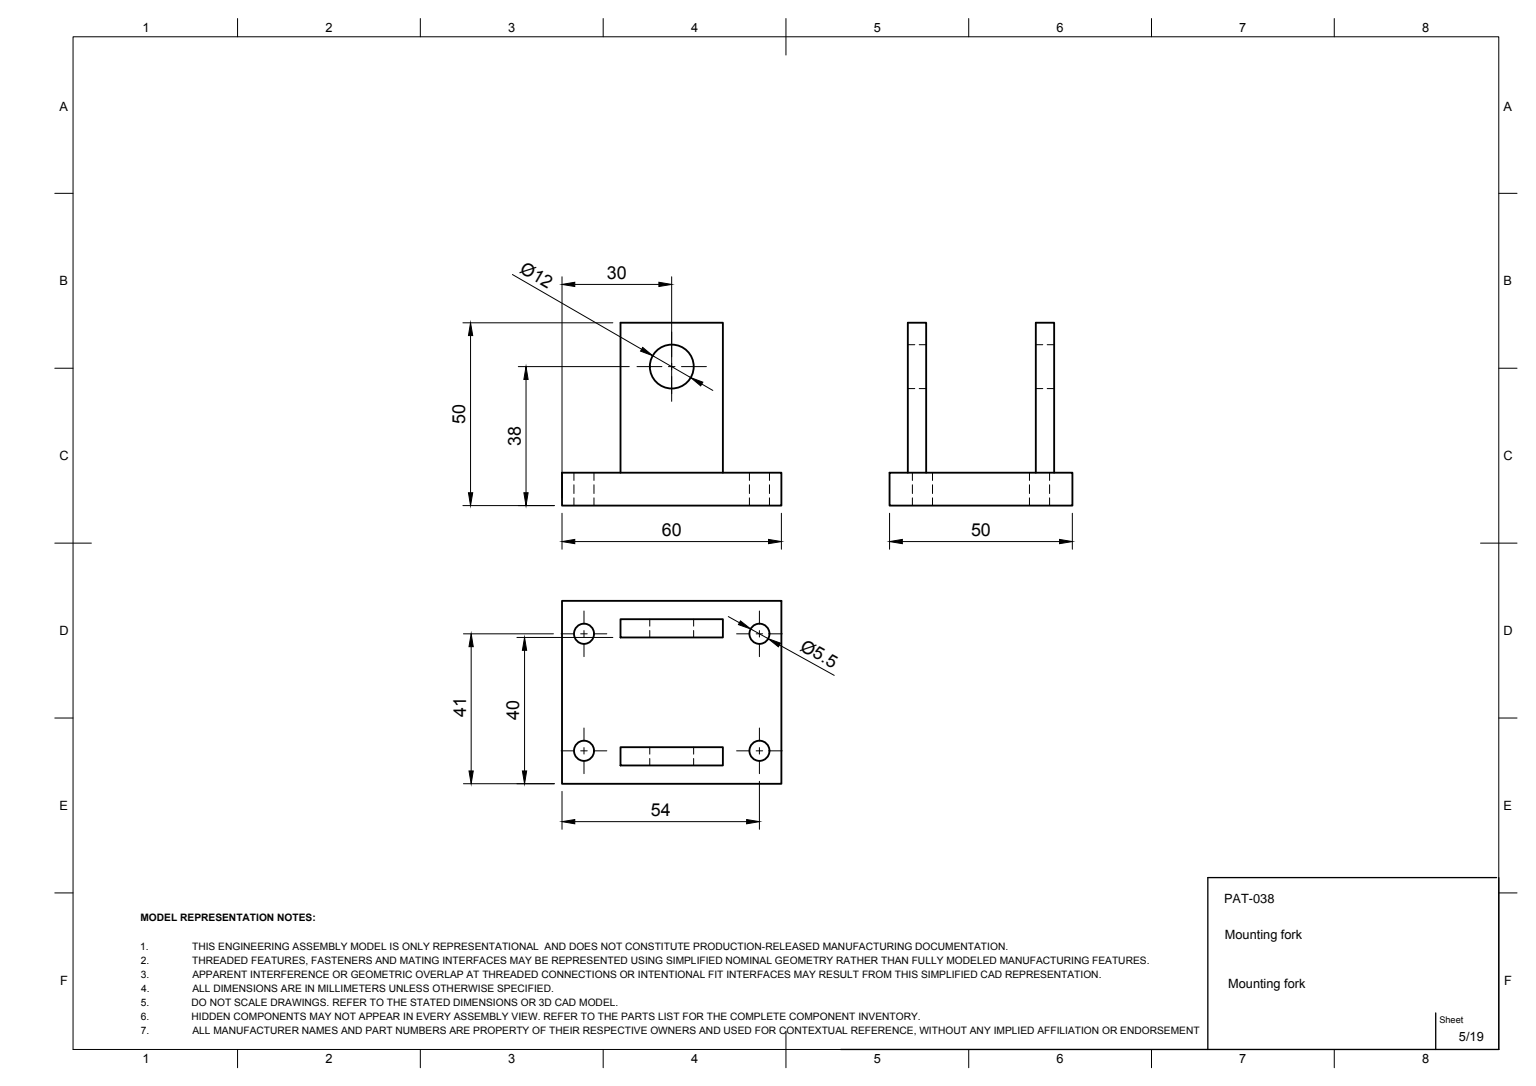
ISO-10303-21;
HEADER;
/* Generated by software containing ST-Developer
 * from STEP Tools, Inc. (www.steptools.com) 
 */

FILE_DESCRIPTION(
/* description */ ('Fork-mounted skate wheel'),
/* implementation_level */ '2;1');

FILE_NAME(
/* name */ 'Mounting fork.step',
/* time_stamp */ '2026-10-29T16:11:26-07:00',
/* author */ (''),
/* organization */ (''),
/* preprocessor_version */ 'ST-DEVELOPER v20.2',
/* originating_system */ 'Autodesk Translation Framework v15.17.0.0',
/* authorisation */ '');

FILE_SCHEMA (('AUTOMOTIVE_DESIGN { 1 0 10303 214 3 1 1 }'));
ENDSEC;

DATA;
#10=MECHANICAL_DESIGN_GEOMETRIC_PRESENTATION_REPRESENTATION('',(#146),#3688);
#122=SHAPE_REPRESENTATION_RELATIONSHIP('SRR','None',#3745,#134);
#134=ADVANCED_BREP_SHAPE_REPRESENTATION('',(#165),#3674);
#146=STYLED_ITEM('',(#3882),#165);
#165=MANIFOLD_SOLID_BREP('Body1',#1807);
#183=FACE_BOUND('',#396,.T.);
#184=FACE_BOUND('',#401,.T.);
#185=FACE_BOUND('',#403,.T.);
#186=FACE_BOUND('',#408,.T.);
#187=FACE_BOUND('',#414,.T.);
#188=FACE_BOUND('',#415,.T.);
#189=FACE_BOUND('',#416,.T.);
#190=FACE_BOUND('',#417,.T.);
#191=FACE_BOUND('',#418,.T.);
#192=FACE_BOUND('',#419,.T.);
#193=FACE_BOUND('',#421,.T.);
#194=FACE_BOUND('',#422,.T.);
#195=FACE_BOUND('',#423,.T.);
#196=FACE_BOUND('',#424,.T.);
#219=PLANE('',#1981);
#220=PLANE('',#1982);
#221=PLANE('',#1983);
#222=PLANE('',#1984);
#223=PLANE('',#1985);
#224=PLANE('',#1986);
#225=PLANE('',#1987);
#226=PLANE('',#1988);
#227=PLANE('',#1989);
#228=PLANE('',#1990);
#229=PLANE('',#1991);
#230=PLANE('',#1992);
#231=PLANE('',#1993);
#232=PLANE('',#1994);
#233=PLANE('',#1995);
#234=PLANE('',#1996);
#276=FACE_OUTER_BOUND('',#389,.T.);
#277=FACE_OUTER_BOUND('',#390,.T.);
#278=FACE_OUTER_BOUND('',#391,.T.);
#279=FACE_OUTER_BOUND('',#392,.T.);
#280=FACE_OUTER_BOUND('',#393,.T.);
#281=FACE_OUTER_BOUND('',#394,.T.);
#282=FACE_OUTER_BOUND('',#395,.T.);
#283=FACE_OUTER_BOUND('',#397,.T.);
#284=FACE_OUTER_BOUND('',#398,.T.);
#285=FACE_OUTER_BOUND('',#399,.T.);
#286=FACE_OUTER_BOUND('',#400,.T.);
#287=FACE_OUTER_BOUND('',#402,.T.);
#288=FACE_OUTER_BOUND('',#404,.T.);
#289=FACE_OUTER_BOUND('',#405,.T.);
#290=FACE_OUTER_BOUND('',#406,.T.);
#291=FACE_OUTER_BOUND('',#407,.T.);
#292=FACE_OUTER_BOUND('',#409,.T.);
#293=FACE_OUTER_BOUND('',#410,.T.);
#294=FACE_OUTER_BOUND('',#411,.T.);
#295=FACE_OUTER_BOUND('',#412,.T.);
#296=FACE_OUTER_BOUND('',#413,.T.);
#297=FACE_OUTER_BOUND('',#420,.T.);
#389=EDGE_LOOP('',(#1217,#1218,#1219,#1220));
#390=EDGE_LOOP('',(#1221,#1222,#1223,#1224));
#391=EDGE_LOOP('',(#1225,#1226,#1227,#1228));
#392=EDGE_LOOP('',(#1229,#1230,#1231,#1232));
#393=EDGE_LOOP('',(#1233,#1234,#1235,#1236));
#394=EDGE_LOOP('',(#1237,#1238,#1239,#1240));
#395=EDGE_LOOP('',(#1241,#1242,#1243,#1244));
#396=EDGE_LOOP('',(#1245));
#397=EDGE_LOOP('',(#1246,#1247,#1248,#1249));
#398=EDGE_LOOP('',(#1250,#1251,#1252,#1253));
#399=EDGE_LOOP('',(#1254,#1255,#1256,#1257));
#400=EDGE_LOOP('',(#1258,#1259,#1260,#1261));
#401=EDGE_LOOP('',(#1262));
#402=EDGE_LOOP('',(#1263,#1264,#1265,#1266));
#403=EDGE_LOOP('',(#1267));
#404=EDGE_LOOP('',(#1268,#1269,#1270,#1271));
#405=EDGE_LOOP('',(#1272,#1273,#1274,#1275));
#406=EDGE_LOOP('',(#1276,#1277,#1278,#1279));
#407=EDGE_LOOP('',(#1280,#1281,#1282,#1283));
#408=EDGE_LOOP('',(#1284));
#409=EDGE_LOOP('',(#1285,#1286,#1287,#1288));
#410=EDGE_LOOP('',(#1289,#1290,#1291,#1292));
#411=EDGE_LOOP('',(#1293,#1294,#1295,#1296));
#412=EDGE_LOOP('',(#1297,#1298,#1299,#1300));
#413=EDGE_LOOP('',(#1301,#1302,#1303,#1304));
#414=EDGE_LOOP('',(#1305,#1306,#1307,#1308));
#415=EDGE_LOOP('',(#1309,#1310,#1311,#1312));
#416=EDGE_LOOP('',(#1313));
#417=EDGE_LOOP('',(#1314));
#418=EDGE_LOOP('',(#1315));
#419=EDGE_LOOP('',(#1316));
#420=EDGE_LOOP('',(#1317,#1318,#1319,#1320));
#421=EDGE_LOOP('',(#1321));
#422=EDGE_LOOP('',(#1322));
#423=EDGE_LOOP('',(#1323));
#424=EDGE_LOOP('',(#1324));
#538=LINE('',#2844,#632);
#539=LINE('',#2850,#633);
#540=LINE('',#2856,#634);
#541=LINE('',#2862,#635);
#542=LINE('',#2868,#636);
#543=LINE('',#2874,#637);
#544=LINE('',#2879,#638);
#545=LINE('',#2881,#639);
#546=LINE('',#2883,#640);
#547=LINE('',#2884,#641);
#548=LINE('',#2887,#642);
#549=LINE('',#2889,#643);
#550=LINE('',#2890,#644);
#551=LINE('',#2893,#645);
#552=LINE('',#2895,#646);
#553=LINE('',#2896,#647);
#554=LINE('',#2898,#648);
#555=LINE('',#2900,#649);
#556=LINE('',#2904,#650);
#557=LINE('',#2906,#651);
#558=LINE('',#2908,#652);
#559=LINE('',#2909,#653);
#560=LINE('',#2912,#654);
#561=LINE('',#2914,#655);
#562=LINE('',#2915,#656);
#563=LINE('',#2918,#657);
#564=LINE('',#2920,#658);
#565=LINE('',#2921,#659);
#566=LINE('',#2923,#660);
#567=LINE('',#2925,#661);
#568=LINE('',#2929,#662);
#569=LINE('',#2931,#663);
#570=LINE('',#2933,#664);
#571=LINE('',#2934,#665);
#572=LINE('',#2937,#666);
#573=LINE('',#2939,#667);
#574=LINE('',#2940,#668);
#575=LINE('',#2943,#669);
#576=LINE('',#2945,#670);
#577=LINE('',#2946,#671);
#578=LINE('',#2948,#672);
#579=LINE('',#2949,#673);
#632=VECTOR('',#2231,0.275);
#633=VECTOR('',#2238,0.275);
#634=VECTOR('',#2245,0.275);
#635=VECTOR('',#2252,0.275);
#636=VECTOR('',#2259,0.6);
#637=VECTOR('',#2266,0.6);
#638=VECTOR('',#2271,1.);
#639=VECTOR('',#2272,1.);
#640=VECTOR('',#2273,1.);
#641=VECTOR('',#2274,1.);
#642=VECTOR('',#2277,1.);
#643=VECTOR('',#2278,1.);
#644=VECTOR('',#2279,1.);
#645=VECTOR('',#2282,1.);
#646=VECTOR('',#2283,1.);
#647=VECTOR('',#2284,1.);
#648=VECTOR('',#2287,1.);
#649=VECTOR('',#2290,1.);
#650=VECTOR('',#2293,1.);
#651=VECTOR('',#2294,1.);
#652=VECTOR('',#2295,1.);
#653=VECTOR('',#2296,1.);
#654=VECTOR('',#2299,1.);
#655=VECTOR('',#2300,1.);
#656=VECTOR('',#2301,1.);
#657=VECTOR('',#2304,1.);
#658=VECTOR('',#2305,1.);
#659=VECTOR('',#2306,1.);
#660=VECTOR('',#2309,1.);
#661=VECTOR('',#2312,1.);
#662=VECTOR('',#2315,1.);
#663=VECTOR('',#2316,1.);
#664=VECTOR('',#2317,1.);
#665=VECTOR('',#2318,1.);
#666=VECTOR('',#2321,1.);
#667=VECTOR('',#2322,1.);
#668=VECTOR('',#2323,1.);
#669=VECTOR('',#2326,1.);
#670=VECTOR('',#2327,1.);
#671=VECTOR('',#2328,1.);
#672=VECTOR('',#2331,1.);
#673=VECTOR('',#2332,1.);
#726=CIRCLE('',#1964,0.275);
#727=CIRCLE('',#1965,0.275);
#728=CIRCLE('',#1967,0.275);
#729=CIRCLE('',#1968,0.275);
#730=CIRCLE('',#1970,0.275);
#731=CIRCLE('',#1971,0.275);
#732=CIRCLE('',#1973,0.275);
#733=CIRCLE('',#1974,0.275);
#734=CIRCLE('',#1976,0.6);
#735=CIRCLE('',#1977,0.6);
#736=CIRCLE('',#1979,0.6);
#737=CIRCLE('',#1980,0.6);
#840=VERTEX_POINT('',#2841);
#841=VERTEX_POINT('',#2843);
#842=VERTEX_POINT('',#2847);
#843=VERTEX_POINT('',#2849);
#844=VERTEX_POINT('',#2853);
#845=VERTEX_POINT('',#2855);
#846=VERTEX_POINT('',#2859);
#847=VERTEX_POINT('',#2861);
#848=VERTEX_POINT('',#2865);
#849=VERTEX_POINT('',#2867);
#850=VERTEX_POINT('',#2871);
#851=VERTEX_POINT('',#2873);
#852=VERTEX_POINT('',#2877);
#853=VERTEX_POINT('',#2878);
#854=VERTEX_POINT('',#2880);
#855=VERTEX_POINT('',#2882);
#856=VERTEX_POINT('',#2886);
#857=VERTEX_POINT('',#2888);
#858=VERTEX_POINT('',#2892);
#859=VERTEX_POINT('',#2894);
#860=VERTEX_POINT('',#2902);
#861=VERTEX_POINT('',#2903);
#862=VERTEX_POINT('',#2905);
#863=VERTEX_POINT('',#2907);
#864=VERTEX_POINT('',#2911);
#865=VERTEX_POINT('',#2913);
#866=VERTEX_POINT('',#2917);
#867=VERTEX_POINT('',#2919);
#868=VERTEX_POINT('',#2927);
#869=VERTEX_POINT('',#2928);
#870=VERTEX_POINT('',#2930);
#871=VERTEX_POINT('',#2932);
#872=VERTEX_POINT('',#2936);
#873=VERTEX_POINT('',#2938);
#874=VERTEX_POINT('',#2942);
#875=VERTEX_POINT('',#2944);
#995=EDGE_CURVE('',#840,#840,#726,.T.);
#996=EDGE_CURVE('',#840,#841,#538,.T.);
#997=EDGE_CURVE('',#841,#841,#727,.T.);
#998=EDGE_CURVE('',#842,#842,#728,.T.);
#999=EDGE_CURVE('',#842,#843,#539,.T.);
#1000=EDGE_CURVE('',#843,#843,#729,.T.);
#1001=EDGE_CURVE('',#844,#844,#730,.T.);
#1002=EDGE_CURVE('',#844,#845,#540,.T.);
#1003=EDGE_CURVE('',#845,#845,#731,.T.);
#1004=EDGE_CURVE('',#846,#846,#732,.T.);
#1005=EDGE_CURVE('',#846,#847,#541,.T.);
#1006=EDGE_CURVE('',#847,#847,#733,.T.);
#1007=EDGE_CURVE('',#848,#848,#734,.T.);
#1008=EDGE_CURVE('',#848,#849,#542,.T.);
#1009=EDGE_CURVE('',#849,#849,#735,.T.);
#1010=EDGE_CURVE('',#850,#850,#736,.T.);
#1011=EDGE_CURVE('',#850,#851,#543,.T.);
#1012=EDGE_CURVE('',#851,#851,#737,.T.);
#1013=EDGE_CURVE('',#852,#853,#544,.T.);
#1014=EDGE_CURVE('',#852,#854,#545,.T.);
#1015=EDGE_CURVE('',#854,#855,#546,.T.);
#1016=EDGE_CURVE('',#855,#853,#547,.T.);
#1017=EDGE_CURVE('',#856,#852,#548,.T.);
#1018=EDGE_CURVE('',#857,#856,#549,.T.);
#1019=EDGE_CURVE('',#854,#857,#550,.T.);
#1020=EDGE_CURVE('',#853,#858,#551,.T.);
#1021=EDGE_CURVE('',#855,#859,#552,.T.);
#1022=EDGE_CURVE('',#858,#859,#553,.T.);
#1023=EDGE_CURVE('',#859,#857,#554,.T.);
#1024=EDGE_CURVE('',#858,#856,#555,.T.);
#1025=EDGE_CURVE('',#860,#861,#556,.T.);
#1026=EDGE_CURVE('',#860,#862,#557,.T.);
#1027=EDGE_CURVE('',#862,#863,#558,.T.);
#1028=EDGE_CURVE('',#863,#861,#559,.T.);
#1029=EDGE_CURVE('',#864,#860,#560,.T.);
#1030=EDGE_CURVE('',#865,#864,#561,.T.);
#1031=EDGE_CURVE('',#862,#865,#562,.T.);
#1032=EDGE_CURVE('',#861,#866,#563,.T.);
#1033=EDGE_CURVE('',#863,#867,#564,.T.);
#1034=EDGE_CURVE('',#866,#867,#565,.T.);
#1035=EDGE_CURVE('',#867,#865,#566,.T.);
#1036=EDGE_CURVE('',#866,#864,#567,.T.);
#1037=EDGE_CURVE('',#868,#869,#568,.T.);
#1038=EDGE_CURVE('',#869,#870,#569,.T.);
#1039=EDGE_CURVE('',#871,#870,#570,.T.);
#1040=EDGE_CURVE('',#868,#871,#571,.T.);
#1041=EDGE_CURVE('',#872,#868,#572,.T.);
#1042=EDGE_CURVE('',#873,#871,#573,.T.);
#1043=EDGE_CURVE('',#872,#873,#574,.T.);
#1044=EDGE_CURVE('',#874,#872,#575,.T.);
#1045=EDGE_CURVE('',#875,#873,#576,.T.);
#1046=EDGE_CURVE('',#874,#875,#577,.T.);
#1047=EDGE_CURVE('',#869,#874,#578,.T.);
#1048=EDGE_CURVE('',#870,#875,#579,.T.);
#1217=ORIENTED_EDGE('',*,*,#995,.F.);
#1218=ORIENTED_EDGE('',*,*,#996,.T.);
#1219=ORIENTED_EDGE('',*,*,#997,.F.);
#1220=ORIENTED_EDGE('',*,*,#996,.F.);
#1221=ORIENTED_EDGE('',*,*,#998,.F.);
#1222=ORIENTED_EDGE('',*,*,#999,.T.);
#1223=ORIENTED_EDGE('',*,*,#1000,.F.);
#1224=ORIENTED_EDGE('',*,*,#999,.F.);
#1225=ORIENTED_EDGE('',*,*,#1001,.F.);
#1226=ORIENTED_EDGE('',*,*,#1002,.T.);
#1227=ORIENTED_EDGE('',*,*,#1003,.F.);
#1228=ORIENTED_EDGE('',*,*,#1002,.F.);
#1229=ORIENTED_EDGE('',*,*,#1004,.F.);
#1230=ORIENTED_EDGE('',*,*,#1005,.T.);
#1231=ORIENTED_EDGE('',*,*,#1006,.F.);
#1232=ORIENTED_EDGE('',*,*,#1005,.F.);
#1233=ORIENTED_EDGE('',*,*,#1007,.F.);
#1234=ORIENTED_EDGE('',*,*,#1008,.T.);
#1235=ORIENTED_EDGE('',*,*,#1009,.F.);
#1236=ORIENTED_EDGE('',*,*,#1008,.F.);
#1237=ORIENTED_EDGE('',*,*,#1010,.F.);
#1238=ORIENTED_EDGE('',*,*,#1011,.T.);
#1239=ORIENTED_EDGE('',*,*,#1012,.F.);
#1240=ORIENTED_EDGE('',*,*,#1011,.F.);
#1241=ORIENTED_EDGE('',*,*,#1013,.F.);
#1242=ORIENTED_EDGE('',*,*,#1014,.T.);
#1243=ORIENTED_EDGE('',*,*,#1015,.T.);
#1244=ORIENTED_EDGE('',*,*,#1016,.T.);
#1245=ORIENTED_EDGE('',*,*,#1010,.T.);
#1246=ORIENTED_EDGE('',*,*,#1017,.F.);
#1247=ORIENTED_EDGE('',*,*,#1018,.F.);
#1248=ORIENTED_EDGE('',*,*,#1019,.F.);
#1249=ORIENTED_EDGE('',*,*,#1014,.F.);
#1250=ORIENTED_EDGE('',*,*,#1020,.F.);
#1251=ORIENTED_EDGE('',*,*,#1016,.F.);
#1252=ORIENTED_EDGE('',*,*,#1021,.T.);
#1253=ORIENTED_EDGE('',*,*,#1022,.F.);
#1254=ORIENTED_EDGE('',*,*,#1015,.F.);
#1255=ORIENTED_EDGE('',*,*,#1019,.T.);
#1256=ORIENTED_EDGE('',*,*,#1023,.F.);
#1257=ORIENTED_EDGE('',*,*,#1021,.F.);
#1258=ORIENTED_EDGE('',*,*,#1024,.F.);
#1259=ORIENTED_EDGE('',*,*,#1022,.T.);
#1260=ORIENTED_EDGE('',*,*,#1023,.T.);
#1261=ORIENTED_EDGE('',*,*,#1018,.T.);
#1262=ORIENTED_EDGE('',*,*,#1012,.T.);
#1263=ORIENTED_EDGE('',*,*,#1025,.F.);
#1264=ORIENTED_EDGE('',*,*,#1026,.T.);
#1265=ORIENTED_EDGE('',*,*,#1027,.T.);
#1266=ORIENTED_EDGE('',*,*,#1028,.T.);
#1267=ORIENTED_EDGE('',*,*,#1007,.T.);
#1268=ORIENTED_EDGE('',*,*,#1029,.F.);
#1269=ORIENTED_EDGE('',*,*,#1030,.F.);
#1270=ORIENTED_EDGE('',*,*,#1031,.F.);
#1271=ORIENTED_EDGE('',*,*,#1026,.F.);
#1272=ORIENTED_EDGE('',*,*,#1032,.F.);
#1273=ORIENTED_EDGE('',*,*,#1028,.F.);
#1274=ORIENTED_EDGE('',*,*,#1033,.T.);
#1275=ORIENTED_EDGE('',*,*,#1034,.F.);
#1276=ORIENTED_EDGE('',*,*,#1027,.F.);
#1277=ORIENTED_EDGE('',*,*,#1031,.T.);
#1278=ORIENTED_EDGE('',*,*,#1035,.F.);
#1279=ORIENTED_EDGE('',*,*,#1033,.F.);
#1280=ORIENTED_EDGE('',*,*,#1036,.F.);
#1281=ORIENTED_EDGE('',*,*,#1034,.T.);
#1282=ORIENTED_EDGE('',*,*,#1035,.T.);
#1283=ORIENTED_EDGE('',*,*,#1030,.T.);
#1284=ORIENTED_EDGE('',*,*,#1009,.T.);
#1285=ORIENTED_EDGE('',*,*,#1037,.T.);
#1286=ORIENTED_EDGE('',*,*,#1038,.T.);
#1287=ORIENTED_EDGE('',*,*,#1039,.F.);
#1288=ORIENTED_EDGE('',*,*,#1040,.F.);
#1289=ORIENTED_EDGE('',*,*,#1041,.T.);
#1290=ORIENTED_EDGE('',*,*,#1040,.T.);
#1291=ORIENTED_EDGE('',*,*,#1042,.F.);
#1292=ORIENTED_EDGE('',*,*,#1043,.F.);
#1293=ORIENTED_EDGE('',*,*,#1044,.T.);
#1294=ORIENTED_EDGE('',*,*,#1043,.T.);
#1295=ORIENTED_EDGE('',*,*,#1045,.F.);
#1296=ORIENTED_EDGE('',*,*,#1046,.F.);
#1297=ORIENTED_EDGE('',*,*,#1047,.T.);
#1298=ORIENTED_EDGE('',*,*,#1046,.T.);
#1299=ORIENTED_EDGE('',*,*,#1048,.F.);
#1300=ORIENTED_EDGE('',*,*,#1038,.F.);
#1301=ORIENTED_EDGE('',*,*,#1048,.T.);
#1302=ORIENTED_EDGE('',*,*,#1045,.T.);
#1303=ORIENTED_EDGE('',*,*,#1042,.T.);
#1304=ORIENTED_EDGE('',*,*,#1039,.T.);
#1305=ORIENTED_EDGE('',*,*,#1029,.T.);
#1306=ORIENTED_EDGE('',*,*,#1025,.T.);
#1307=ORIENTED_EDGE('',*,*,#1032,.T.);
#1308=ORIENTED_EDGE('',*,*,#1036,.T.);
#1309=ORIENTED_EDGE('',*,*,#1017,.T.);
#1310=ORIENTED_EDGE('',*,*,#1013,.T.);
#1311=ORIENTED_EDGE('',*,*,#1020,.T.);
#1312=ORIENTED_EDGE('',*,*,#1024,.T.);
#1313=ORIENTED_EDGE('',*,*,#1006,.T.);
#1314=ORIENTED_EDGE('',*,*,#1003,.T.);
#1315=ORIENTED_EDGE('',*,*,#1000,.T.);
#1316=ORIENTED_EDGE('',*,*,#997,.T.);
#1317=ORIENTED_EDGE('',*,*,#1047,.F.);
#1318=ORIENTED_EDGE('',*,*,#1037,.F.);
#1319=ORIENTED_EDGE('',*,*,#1041,.F.);
#1320=ORIENTED_EDGE('',*,*,#1044,.F.);
#1321=ORIENTED_EDGE('',*,*,#995,.T.);
#1322=ORIENTED_EDGE('',*,*,#998,.T.);
#1323=ORIENTED_EDGE('',*,*,#1001,.T.);
#1324=ORIENTED_EDGE('',*,*,#1004,.T.);
#1661=CYLINDRICAL_SURFACE('',#1963,0.275);
#1662=CYLINDRICAL_SURFACE('',#1966,0.275);
#1663=CYLINDRICAL_SURFACE('',#1969,0.275);
#1664=CYLINDRICAL_SURFACE('',#1972,0.275);
#1665=CYLINDRICAL_SURFACE('',#1975,0.6);
#1666=CYLINDRICAL_SURFACE('',#1978,0.6);
#1694=ADVANCED_FACE('',(#276),#1661,.F.);
#1695=ADVANCED_FACE('',(#277),#1662,.F.);
#1696=ADVANCED_FACE('',(#278),#1663,.F.);
#1697=ADVANCED_FACE('',(#279),#1664,.F.);
#1698=ADVANCED_FACE('',(#280),#1665,.F.);
#1699=ADVANCED_FACE('',(#281),#1666,.F.);
#1700=ADVANCED_FACE('',(#282,#183),#219,.F.);
#1701=ADVANCED_FACE('',(#283),#220,.T.);
#1702=ADVANCED_FACE('',(#284),#221,.T.);
#1703=ADVANCED_FACE('',(#285),#222,.T.);
#1704=ADVANCED_FACE('',(#286,#184),#223,.T.);
#1705=ADVANCED_FACE('',(#287,#185),#224,.F.);
#1706=ADVANCED_FACE('',(#288),#225,.T.);
#1707=ADVANCED_FACE('',(#289),#226,.T.);
#1708=ADVANCED_FACE('',(#290),#227,.T.);
#1709=ADVANCED_FACE('',(#291,#186),#228,.T.);
#1710=ADVANCED_FACE('',(#292),#229,.T.);
#1711=ADVANCED_FACE('',(#293),#230,.T.);
#1712=ADVANCED_FACE('',(#294),#231,.T.);
#1713=ADVANCED_FACE('',(#295),#232,.T.);
#1714=ADVANCED_FACE('',(#296,#187,#188,#189,#190,#191,#192),#233,.T.);
#1715=ADVANCED_FACE('',(#297,#193,#194,#195,#196),#234,.F.);
#1807=CLOSED_SHELL('',(#1694,#1695,#1696,#1697,#1698,#1699,#1700,#1701,
#1702,#1703,#1704,#1705,#1706,#1707,#1708,#1709,#1710,#1711,#1712,#1713,
#1714,#1715));
#1962=AXIS2_PLACEMENT_3D('',#2839,#2225,#2226);
#1963=AXIS2_PLACEMENT_3D('',#2840,#2227,#2228);
#1964=AXIS2_PLACEMENT_3D('',#2842,#2229,#2230);
#1965=AXIS2_PLACEMENT_3D('',#2845,#2232,#2233);
#1966=AXIS2_PLACEMENT_3D('',#2846,#2234,#2235);
#1967=AXIS2_PLACEMENT_3D('',#2848,#2236,#2237);
#1968=AXIS2_PLACEMENT_3D('',#2851,#2239,#2240);
#1969=AXIS2_PLACEMENT_3D('',#2852,#2241,#2242);
#1970=AXIS2_PLACEMENT_3D('',#2854,#2243,#2244);
#1971=AXIS2_PLACEMENT_3D('',#2857,#2246,#2247);
#1972=AXIS2_PLACEMENT_3D('',#2858,#2248,#2249);
#1973=AXIS2_PLACEMENT_3D('',#2860,#2250,#2251);
#1974=AXIS2_PLACEMENT_3D('',#2863,#2253,#2254);
#1975=AXIS2_PLACEMENT_3D('',#2864,#2255,#2256);
#1976=AXIS2_PLACEMENT_3D('',#2866,#2257,#2258);
#1977=AXIS2_PLACEMENT_3D('',#2869,#2260,#2261);
#1978=AXIS2_PLACEMENT_3D('',#2870,#2262,#2263);
#1979=AXIS2_PLACEMENT_3D('',#2872,#2264,#2265);
#1980=AXIS2_PLACEMENT_3D('',#2875,#2267,#2268);
#1981=AXIS2_PLACEMENT_3D('',#2876,#2269,#2270);
#1982=AXIS2_PLACEMENT_3D('',#2885,#2275,#2276);
#1983=AXIS2_PLACEMENT_3D('',#2891,#2280,#2281);
#1984=AXIS2_PLACEMENT_3D('',#2897,#2285,#2286);
#1985=AXIS2_PLACEMENT_3D('',#2899,#2288,#2289);
#1986=AXIS2_PLACEMENT_3D('',#2901,#2291,#2292);
#1987=AXIS2_PLACEMENT_3D('',#2910,#2297,#2298);
#1988=AXIS2_PLACEMENT_3D('',#2916,#2302,#2303);
#1989=AXIS2_PLACEMENT_3D('',#2922,#2307,#2308);
#1990=AXIS2_PLACEMENT_3D('',#2924,#2310,#2311);
#1991=AXIS2_PLACEMENT_3D('',#2926,#2313,#2314);
#1992=AXIS2_PLACEMENT_3D('',#2935,#2319,#2320);
#1993=AXIS2_PLACEMENT_3D('',#2941,#2324,#2325);
#1994=AXIS2_PLACEMENT_3D('',#2947,#2329,#2330);
#1995=AXIS2_PLACEMENT_3D('',#2950,#2333,#2334);
#1996=AXIS2_PLACEMENT_3D('',#2951,#2335,#2336);
#2225=DIRECTION('axis',(0.,0.,1.));
#2226=DIRECTION('refdir',(1.,0.,0.));
#2227=DIRECTION('center_axis',(0.,0.,1.));
#2228=DIRECTION('ref_axis',(1.,0.,0.));
#2229=DIRECTION('center_axis',(0.,0.,1.));
#2230=DIRECTION('ref_axis',(1.,0.,0.));
#2231=DIRECTION('',(0.,0.,1.));
#2232=DIRECTION('center_axis',(0.,0.,-1.));
#2233=DIRECTION('ref_axis',(1.,0.,0.));
#2234=DIRECTION('center_axis',(0.,0.,1.));
#2235=DIRECTION('ref_axis',(1.,0.,0.));
#2236=DIRECTION('center_axis',(0.,0.,1.));
#2237=DIRECTION('ref_axis',(1.,0.,0.));
#2238=DIRECTION('',(0.,0.,1.));
#2239=DIRECTION('center_axis',(0.,0.,-1.));
#2240=DIRECTION('ref_axis',(1.,0.,0.));
#2241=DIRECTION('center_axis',(0.,0.,1.));
#2242=DIRECTION('ref_axis',(1.,0.,0.));
#2243=DIRECTION('center_axis',(0.,0.,1.));
#2244=DIRECTION('ref_axis',(1.,0.,0.));
#2245=DIRECTION('',(0.,0.,1.));
#2246=DIRECTION('center_axis',(0.,0.,-1.));
#2247=DIRECTION('ref_axis',(1.,0.,0.));
#2248=DIRECTION('center_axis',(0.,0.,1.));
#2249=DIRECTION('ref_axis',(1.,0.,0.));
#2250=DIRECTION('center_axis',(0.,0.,1.));
#2251=DIRECTION('ref_axis',(1.,0.,0.));
#2252=DIRECTION('',(0.,0.,1.));
#2253=DIRECTION('center_axis',(0.,0.,-1.));
#2254=DIRECTION('ref_axis',(1.,0.,0.));
#2255=DIRECTION('center_axis',(0.,1.,0.));
#2256=DIRECTION('ref_axis',(1.,0.,0.));
#2257=DIRECTION('center_axis',(0.,1.,0.));
#2258=DIRECTION('ref_axis',(1.,0.,0.));
#2259=DIRECTION('',(0.,1.,0.));
#2260=DIRECTION('center_axis',(0.,-1.,0.));
#2261=DIRECTION('ref_axis',(1.,0.,0.));
#2262=DIRECTION('center_axis',(0.,1.,0.));
#2263=DIRECTION('ref_axis',(1.,0.,0.));
#2264=DIRECTION('center_axis',(0.,1.,0.));
#2265=DIRECTION('ref_axis',(1.,0.,0.));
#2266=DIRECTION('',(0.,1.,0.));
#2267=DIRECTION('center_axis',(0.,-1.,0.));
#2268=DIRECTION('ref_axis',(1.,0.,0.));
#2269=DIRECTION('center_axis',(0.,1.,0.));
#2270=DIRECTION('ref_axis',(1.,0.,0.));
#2271=DIRECTION('',(-1.,0.,0.));
#2272=DIRECTION('',(0.,0.,1.));
#2273=DIRECTION('',(-1.,0.,0.));
#2274=DIRECTION('',(0.,0.,-1.));
#2275=DIRECTION('center_axis',(1.,0.,0.));
#2276=DIRECTION('ref_axis',(0.,0.,-1.));
#2277=DIRECTION('',(0.,-1.,0.));
#2278=DIRECTION('',(0.,0.,-1.));
#2279=DIRECTION('',(0.,1.,0.));
#2280=DIRECTION('center_axis',(-1.,0.,0.));
#2281=DIRECTION('ref_axis',(0.,0.,1.));
#2282=DIRECTION('',(0.,1.,0.));
#2283=DIRECTION('',(0.,1.,0.));
#2284=DIRECTION('',(0.,0.,1.));
#2285=DIRECTION('center_axis',(0.,0.,1.));
#2286=DIRECTION('ref_axis',(1.,0.,0.));
#2287=DIRECTION('',(1.,0.,0.));
#2288=DIRECTION('center_axis',(0.,1.,0.));
#2289=DIRECTION('ref_axis',(0.,0.,1.));
#2290=DIRECTION('',(1.,0.,0.));
#2291=DIRECTION('center_axis',(0.,1.,0.));
#2292=DIRECTION('ref_axis',(1.,0.,0.));
#2293=DIRECTION('',(-1.,0.,0.));
#2294=DIRECTION('',(0.,0.,1.));
#2295=DIRECTION('',(-1.,0.,0.));
#2296=DIRECTION('',(0.,0.,-1.));
#2297=DIRECTION('center_axis',(1.,0.,0.));
#2298=DIRECTION('ref_axis',(0.,0.,-1.));
#2299=DIRECTION('',(0.,-1.,0.));
#2300=DIRECTION('',(0.,0.,-1.));
#2301=DIRECTION('',(0.,1.,0.));
#2302=DIRECTION('center_axis',(-1.,0.,0.));
#2303=DIRECTION('ref_axis',(0.,0.,1.));
#2304=DIRECTION('',(0.,1.,0.));
#2305=DIRECTION('',(0.,1.,0.));
#2306=DIRECTION('',(0.,0.,1.));
#2307=DIRECTION('center_axis',(0.,0.,1.));
#2308=DIRECTION('ref_axis',(1.,0.,0.));
#2309=DIRECTION('',(1.,0.,0.));
#2310=DIRECTION('center_axis',(0.,1.,0.));
#2311=DIRECTION('ref_axis',(0.,0.,1.));
#2312=DIRECTION('',(1.,0.,0.));
#2313=DIRECTION('center_axis',(0.,1.,0.));
#2314=DIRECTION('ref_axis',(-1.,0.,0.));
#2315=DIRECTION('',(-1.,0.,0.));
#2316=DIRECTION('',(0.,0.,1.));
#2317=DIRECTION('',(-1.,0.,0.));
#2318=DIRECTION('',(0.,0.,1.));
#2319=DIRECTION('center_axis',(1.,0.,0.));
#2320=DIRECTION('ref_axis',(0.,1.,0.));
#2321=DIRECTION('',(0.,1.,0.));
#2322=DIRECTION('',(0.,1.,0.));
#2323=DIRECTION('',(0.,0.,1.));
#2324=DIRECTION('center_axis',(0.,-1.,0.));
#2325=DIRECTION('ref_axis',(1.,0.,0.));
#2326=DIRECTION('',(1.,0.,0.));
#2327=DIRECTION('',(1.,0.,0.));
#2328=DIRECTION('',(0.,0.,1.));
#2329=DIRECTION('center_axis',(-1.,0.,0.));
#2330=DIRECTION('ref_axis',(0.,-1.,0.));
#2331=DIRECTION('',(0.,-1.,0.));
#2332=DIRECTION('',(0.,-1.,0.));
#2333=DIRECTION('center_axis',(0.,0.,1.));
#2334=DIRECTION('ref_axis',(1.,0.,0.));
#2335=DIRECTION('center_axis',(0.,0.,1.));
#2336=DIRECTION('ref_axis',(1.,0.,0.));
#2839=CARTESIAN_POINT('',(0.,0.,0.));
#2840=CARTESIAN_POINT('Origin',(2.4,-1.6,-0.1));
#2841=CARTESIAN_POINT('',(2.125,-1.6,-0.3));
#2842=CARTESIAN_POINT('Origin',(2.4,-1.6,-0.3));
#2843=CARTESIAN_POINT('',(2.125,-1.6,0.6));
#2844=CARTESIAN_POINT('',(2.125,-1.6,-0.1));
#2845=CARTESIAN_POINT('Origin',(2.4,-1.6,0.6));
#2846=CARTESIAN_POINT('Origin',(-2.4,1.6,-0.1));
#2847=CARTESIAN_POINT('',(-2.675,1.6,-0.3));
#2848=CARTESIAN_POINT('Origin',(-2.4,1.6,-0.3));
#2849=CARTESIAN_POINT('',(-2.675,1.6,0.6));
#2850=CARTESIAN_POINT('',(-2.675,1.6,-0.1));
#2851=CARTESIAN_POINT('Origin',(-2.4,1.6,0.6));
#2852=CARTESIAN_POINT('Origin',(-2.4,-1.6,-0.1));
#2853=CARTESIAN_POINT('',(-2.675,-1.6,-0.3));
#2854=CARTESIAN_POINT('Origin',(-2.4,-1.6,-0.3));
#2855=CARTESIAN_POINT('',(-2.675,-1.6,0.6));
#2856=CARTESIAN_POINT('',(-2.675,-1.6,-0.1));
#2857=CARTESIAN_POINT('Origin',(-2.4,-1.6,0.6));
#2858=CARTESIAN_POINT('Origin',(2.4,1.6,-0.1));
#2859=CARTESIAN_POINT('',(2.125,1.6,-0.3));
#2860=CARTESIAN_POINT('Origin',(2.4,1.6,-0.3));
#2861=CARTESIAN_POINT('',(2.125,1.6,0.6));
#2862=CARTESIAN_POINT('',(2.125,1.6,-0.1));
#2863=CARTESIAN_POINT('Origin',(2.4,1.6,0.6));
#2864=CARTESIAN_POINT('Origin',(0.,-2.1,3.5));
#2865=CARTESIAN_POINT('',(-0.6,-2.,3.5));
#2866=CARTESIAN_POINT('Origin',(0.,-2.,3.5));
#2867=CARTESIAN_POINT('',(-0.6,-1.5,3.5));
#2868=CARTESIAN_POINT('',(-0.6,-2.1,3.5));
#2869=CARTESIAN_POINT('Origin',(0.,-1.5,3.5));
#2870=CARTESIAN_POINT('Origin',(0.,-2.1,3.5));
#2871=CARTESIAN_POINT('',(-0.6,1.5,3.5));
#2872=CARTESIAN_POINT('Origin',(0.,1.5,3.5));
#2873=CARTESIAN_POINT('',(-0.6,2.,3.5));
#2874=CARTESIAN_POINT('',(-0.6,-2.1,3.5));
#2875=CARTESIAN_POINT('Origin',(0.,2.,3.5));
#2876=CARTESIAN_POINT('Origin',(0.,1.5,2.6));
#2877=CARTESIAN_POINT('',(1.4,1.5,0.6));
#2878=CARTESIAN_POINT('',(-1.4,1.5,0.600000000000001));
#2879=CARTESIAN_POINT('',(0.,1.5,0.6));
#2880=CARTESIAN_POINT('',(1.4,1.5,4.7));
#2881=CARTESIAN_POINT('',(1.4,1.5,0.5));
#2882=CARTESIAN_POINT('',(-1.4,1.5,4.7));
#2883=CARTESIAN_POINT('',(1.4,1.5,4.7));
#2884=CARTESIAN_POINT('',(-1.4,1.5,4.7));
#2885=CARTESIAN_POINT('Origin',(1.4,1.5,4.7));
#2886=CARTESIAN_POINT('',(1.4,2.,0.6));
#2887=CARTESIAN_POINT('',(1.4,0.75,0.6));
#2888=CARTESIAN_POINT('',(1.4,2.,4.7));
#2889=CARTESIAN_POINT('',(1.4,2.,0.5));
#2890=CARTESIAN_POINT('',(1.4,1.5,4.7));
#2891=CARTESIAN_POINT('Origin',(-1.4,1.5,0.5));
#2892=CARTESIAN_POINT('',(-1.4,2.,0.600000000000001));
#2893=CARTESIAN_POINT('',(-1.4,0.75,0.6));
#2894=CARTESIAN_POINT('',(-1.4,2.,4.7));
#2895=CARTESIAN_POINT('',(-1.4,1.5,4.7));
#2896=CARTESIAN_POINT('',(-1.4,2.,4.7));
#2897=CARTESIAN_POINT('Origin',(-1.4,1.5,4.7));
#2898=CARTESIAN_POINT('',(1.4,2.,4.7));
#2899=CARTESIAN_POINT('Origin',(0.,2.,2.6));
#2900=CARTESIAN_POINT('',(0.,2.,0.6));
#2901=CARTESIAN_POINT('Origin',(0.,-2.,2.6));
#2902=CARTESIAN_POINT('',(1.4,-2.,0.6));
#2903=CARTESIAN_POINT('',(-1.4,-2.,0.600000000000001));
#2904=CARTESIAN_POINT('',(0.,-2.,0.6));
#2905=CARTESIAN_POINT('',(1.4,-2.,4.7));
#2906=CARTESIAN_POINT('',(1.4,-2.,0.5));
#2907=CARTESIAN_POINT('',(-1.4,-2.,4.7));
#2908=CARTESIAN_POINT('',(1.4,-2.,4.7));
#2909=CARTESIAN_POINT('',(-1.4,-2.,4.7));
#2910=CARTESIAN_POINT('Origin',(1.4,-2.,4.7));
#2911=CARTESIAN_POINT('',(1.4,-1.5,0.6));
#2912=CARTESIAN_POINT('',(1.4,-1.,0.6));
#2913=CARTESIAN_POINT('',(1.4,-1.5,4.7));
#2914=CARTESIAN_POINT('',(1.4,-1.5,0.5));
#2915=CARTESIAN_POINT('',(1.4,-2.,4.7));
#2916=CARTESIAN_POINT('Origin',(-1.4,-2.,0.5));
#2917=CARTESIAN_POINT('',(-1.4,-1.5,0.600000000000001));
#2918=CARTESIAN_POINT('',(-1.4,-1.,0.6));
#2919=CARTESIAN_POINT('',(-1.4,-1.5,4.7));
#2920=CARTESIAN_POINT('',(-1.4,-2.,4.7));
#2921=CARTESIAN_POINT('',(-1.4,-1.5,4.7));
#2922=CARTESIAN_POINT('Origin',(-1.4,-2.,4.7));
#2923=CARTESIAN_POINT('',(1.4,-1.5,4.7));
#2924=CARTESIAN_POINT('Origin',(0.,-1.5,2.6));
#2925=CARTESIAN_POINT('',(0.,-1.5,0.6));
#2926=CARTESIAN_POINT('Origin',(3.,2.5,0.));
#2927=CARTESIAN_POINT('',(3.,2.5,-0.3));
#2928=CARTESIAN_POINT('',(-3.,2.5,-0.3));
#2929=CARTESIAN_POINT('',(1.5,2.5,-0.3));
#2930=CARTESIAN_POINT('',(-3.,2.5,0.6));
#2931=CARTESIAN_POINT('',(-3.,2.5,0.));
#2932=CARTESIAN_POINT('',(3.,2.5,0.6));
#2933=CARTESIAN_POINT('',(3.,2.5,0.6));
#2934=CARTESIAN_POINT('',(3.,2.5,0.));
#2935=CARTESIAN_POINT('Origin',(3.,-2.5,0.));
#2936=CARTESIAN_POINT('',(3.,-2.5,-0.3));
#2937=CARTESIAN_POINT('',(3.,-1.25,-0.3));
#2938=CARTESIAN_POINT('',(3.,-2.5,0.6));
#2939=CARTESIAN_POINT('',(3.,-2.5,0.6));
#2940=CARTESIAN_POINT('',(3.,-2.5,0.));
#2941=CARTESIAN_POINT('Origin',(-3.,-2.5,0.));
#2942=CARTESIAN_POINT('',(-3.,-2.5,-0.3));
#2943=CARTESIAN_POINT('',(-1.5,-2.5,-0.3));
#2944=CARTESIAN_POINT('',(-3.,-2.5,0.6));
#2945=CARTESIAN_POINT('',(-3.,-2.5,0.6));
#2946=CARTESIAN_POINT('',(-3.,-2.5,0.));
#2947=CARTESIAN_POINT('Origin',(-3.,2.5,0.));
#2948=CARTESIAN_POINT('',(-3.,1.25,-0.3));
#2949=CARTESIAN_POINT('',(-3.,2.5,0.6));
#2950=CARTESIAN_POINT('Origin',(0.,0.,0.6));
#2951=CARTESIAN_POINT('Origin',(0.,0.,-0.3));
#3657=UNCERTAINTY_MEASURE_WITH_UNIT(LENGTH_MEASURE(0.001),#3689,
'DISTANCE_ACCURACY_VALUE',
'Maximum model space distance between geometric entities at asserted c
onnectivities');
#3671=UNCERTAINTY_MEASURE_WITH_UNIT(LENGTH_MEASURE(0.001),#3689,
'DISTANCE_ACCURACY_VALUE',
'Maximum model space distance between geometric entities at asserted c
onnectivities');
#3674=(
GEOMETRIC_REPRESENTATION_CONTEXT(3)
GLOBAL_UNCERTAINTY_ASSIGNED_CONTEXT((#3657))
GLOBAL_UNIT_ASSIGNED_CONTEXT((#3689,#3691,#3692))
REPRESENTATION_CONTEXT('','3D')
);
#3688=(
GEOMETRIC_REPRESENTATION_CONTEXT(3)
GLOBAL_UNCERTAINTY_ASSIGNED_CONTEXT((#3671))
GLOBAL_UNIT_ASSIGNED_CONTEXT((#3689,#3691,#3692))
REPRESENTATION_CONTEXT('','3D')
);
#3689=(
LENGTH_UNIT()
NAMED_UNIT(*)
SI_UNIT(.CENTI.,.METRE.)
);
#3691=(
NAMED_UNIT(*)
PLANE_ANGLE_UNIT()
SI_UNIT($,.RADIAN.)
);
#3692=(
NAMED_UNIT(*)
SI_UNIT($,.STERADIAN.)
SOLID_ANGLE_UNIT()
);
#3695=SHAPE_DEFINITION_REPRESENTATION(#3711,#3745);
#3711=PRODUCT_DEFINITION_SHAPE('',$,#3762);
#3745=SHAPE_REPRESENTATION('',(#1962),#3674);
#3759=PRODUCT_DEFINITION_CONTEXT('part definition',#3809,'design');
#3762=PRODUCT_DEFINITION('Mounting fork','Mounting fork',#3778,#3759);
#3778=PRODUCT_DEFINITION_FORMATION('',$,#3813);
#3809=APPLICATION_CONTEXT(
'Core Data for Automotive Mechanical Design Process');
#3810=PRODUCT_CONTEXT('part definition',#3809,'mechanical');
#3813=PRODUCT('Mounting fork','Mounting fork','Mounting fork',(#3810));
#3876=COLOUR_RGB('Light Blue',0.38,0.62,0.78);
#3877=FILL_AREA_STYLE_COLOUR('',#3876);
#3878=FILL_AREA_STYLE('',(#3877));
#3879=SURFACE_STYLE_FILL_AREA(#3878);
#3880=SURFACE_SIDE_STYLE('',(#3879));
#3881=SURFACE_STYLE_USAGE(.BOTH.,#3880);
#3882=PRESENTATION_STYLE_ASSIGNMENT((#3881));
ENDSEC;
END-ISO-10303-21;
